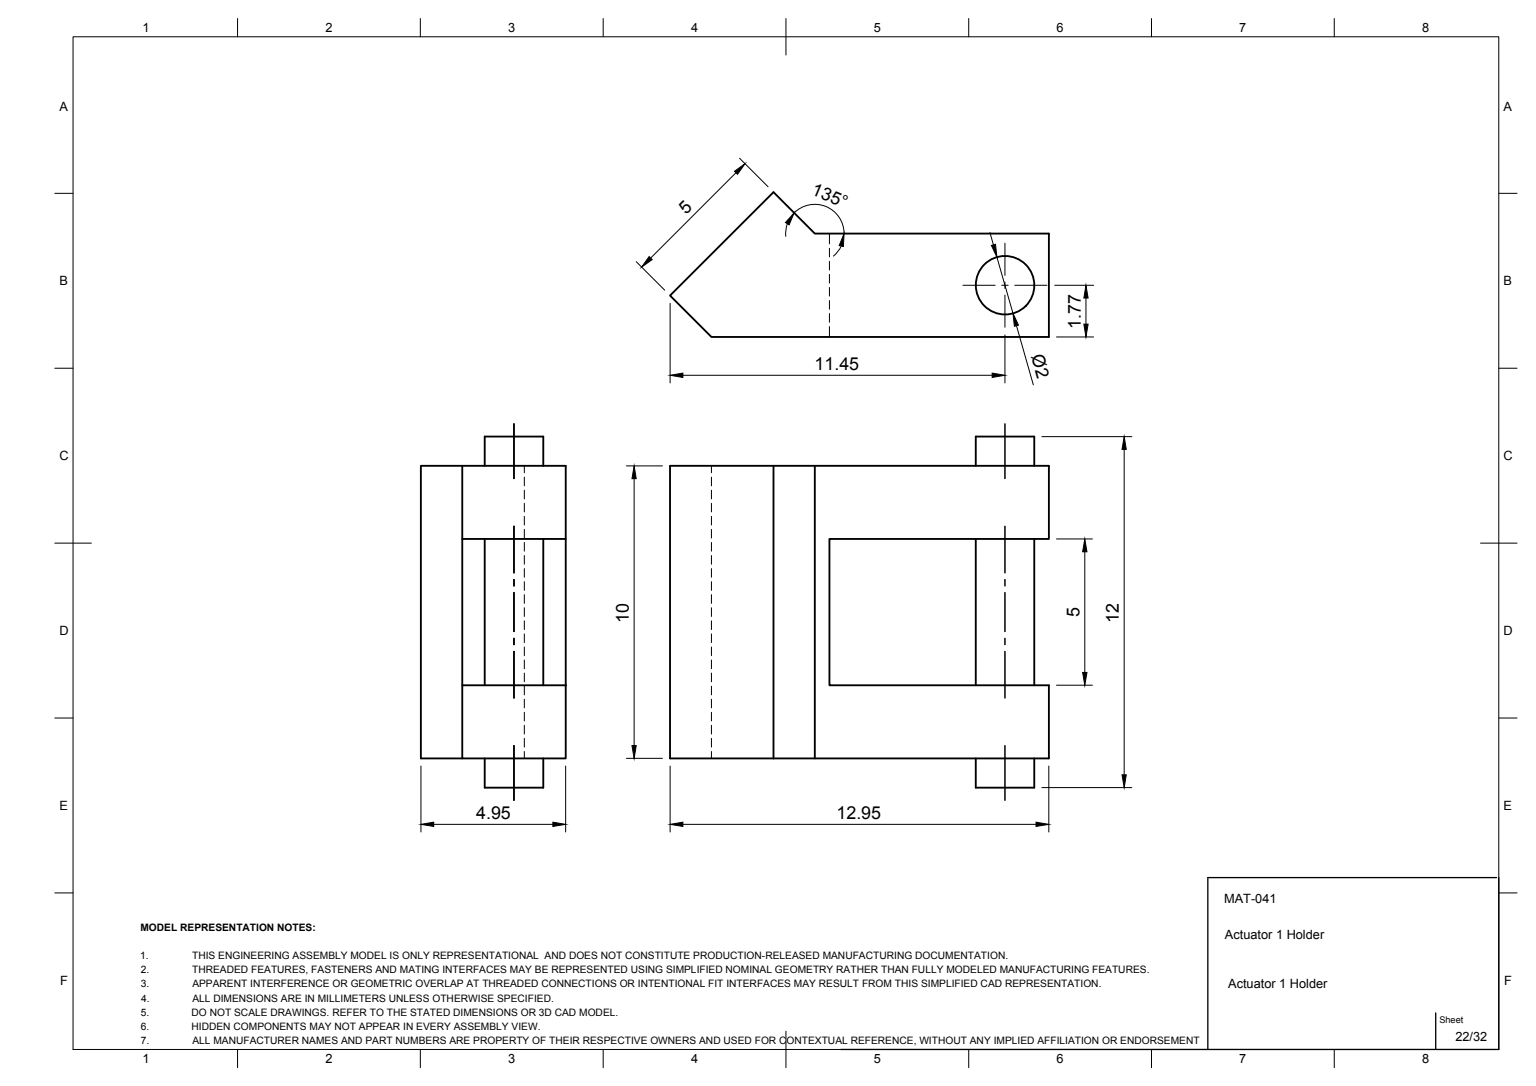
ISO-10303-21;
HEADER;
/* Generated by software containing ST-Developer
 * from STEP Tools, Inc. (www.steptools.com) 
 */

FILE_DESCRIPTION(
/* description */ ('STEP AP214'),
/* implementation_level */ '2;1');

FILE_NAME(
/* name */ 'Actuator 1 Holder.step',
/* time_stamp */ '2026-11-14T21:57:47-08:00',
/* author */ (''),
/* organization */ (''),
/* preprocessor_version */ 'ST-DEVELOPER v20.2',
/* originating_system */ 'Autodesk Translation Framework v15.17.0.0',
/* authorisation */ '');

FILE_SCHEMA (('AUTOMOTIVE_DESIGN { 1 0 10303 214 3 1 1 }'));
ENDSEC;

DATA;
#10=MECHANICAL_DESIGN_GEOMETRIC_PRESENTATION_REPRESENTATION('',(#258),#13199);
#222=SHAPE_REPRESENTATION_RELATIONSHIP('SRR','None',#13293,#240);
#240=ADVANCED_BREP_SHAPE_REPRESENTATION('',(#276),#13189);
#258=STYLED_ITEM('',(#13409),#276);
#276=MANIFOLD_SOLID_BREP('Body1',#6853);
#345=FACE_BOUND('',#2515,.T.);
#346=FACE_BOUND('',#2518,.T.);
#347=FACE_BOUND('',#2525,.T.);
#348=FACE_BOUND('',#2527,.T.);
#524=PLANE('',#7578);
#525=PLANE('',#7579);
#526=PLANE('',#7580);
#527=PLANE('',#7581);
#528=PLANE('',#7582);
#529=PLANE('',#7583);
#530=PLANE('',#7584);
#531=PLANE('',#7585);
#532=PLANE('',#7586);
#533=PLANE('',#7587);
#534=PLANE('',#7588);
#535=PLANE('',#7589);
#536=PLANE('',#7590);
#537=PLANE('',#7591);
#935=LINE('',#11859,#1453);
#936=LINE('',#11865,#1454);
#937=LINE('',#11871,#1455);
#938=LINE('',#11876,#1456);
#939=LINE('',#11878,#1457);
#940=LINE('',#11880,#1458);
#941=LINE('',#11881,#1459);
#942=LINE('',#11885,#1460);
#943=LINE('',#11887,#1461);
#944=LINE('',#11888,#1462);
#945=LINE('',#11890,#1463);
#946=LINE('',#11891,#1464);
#947=LINE('',#11894,#1465);
#948=LINE('',#11896,#1466);
#949=LINE('',#11897,#1467);
#950=LINE('',#11900,#1468);
#951=LINE('',#11902,#1469);
#952=LINE('',#11904,#1470);
#953=LINE('',#11906,#1471);
#954=LINE('',#11907,#1472);
#955=LINE('',#11909,#1473);
#956=LINE('',#11910,#1474);
#957=LINE('',#11914,#1475);
#958=LINE('',#11916,#1476);
#959=LINE('',#11918,#1477);
#960=LINE('',#11919,#1478);
#961=LINE('',#11923,#1479);
#962=LINE('',#11924,#1480);
#963=LINE('',#11926,#1481);
#964=LINE('',#11927,#1482);
#965=LINE('',#11929,#1483);
#966=LINE('',#11931,#1484);
#967=LINE('',#11933,#1485);
#1453=VECTOR('',#9176,1.);
#1454=VECTOR('',#9183,1.);
#1455=VECTOR('',#9190,1.);
#1456=VECTOR('',#9195,1000.);
#1457=VECTOR('',#9196,1000.);
#1458=VECTOR('',#9197,1000.);
#1459=VECTOR('',#9198,1000.);
#1460=VECTOR('',#9201,1000.);
#1461=VECTOR('',#9202,1000.);
#1462=VECTOR('',#9203,1000.);
#1463=VECTOR('',#9204,1000.);
#1464=VECTOR('',#9205,1000.);
#1465=VECTOR('',#9208,1000.);
#1466=VECTOR('',#9209,1000.);
#1467=VECTOR('',#9210,1000.);
#1468=VECTOR('',#9213,1000.);
#1469=VECTOR('',#9214,1000.);
#1470=VECTOR('',#9215,1000.);
#1471=VECTOR('',#9216,1000.);
#1472=VECTOR('',#9217,1000.);
#1473=VECTOR('',#9220,1000.);
#1474=VECTOR('',#9221,1000.);
#1475=VECTOR('',#9226,1000.);
#1476=VECTOR('',#9227,1000.);
#1477=VECTOR('',#9228,1000.);
#1478=VECTOR('',#9229,1000.);
#1479=VECTOR('',#9232,1000.);
#1480=VECTOR('',#9233,1000.);
#1481=VECTOR('',#9234,1000.);
#1482=VECTOR('',#9235,1000.);
#1483=VECTOR('',#9238,1000.);
#1484=VECTOR('',#9241,1000.);
#1485=VECTOR('',#9244,1000.);
#1751=CYLINDRICAL_SURFACE('',#7569,1.);
#1752=CYLINDRICAL_SURFACE('',#7572,1.);
#1753=CYLINDRICAL_SURFACE('',#7575,1.);
#2058=FACE_OUTER_BOUND('',#2510,.T.);
#2059=FACE_OUTER_BOUND('',#2511,.T.);
#2060=FACE_OUTER_BOUND('',#2512,.T.);
#2061=FACE_OUTER_BOUND('',#2513,.T.);
#2062=FACE_OUTER_BOUND('',#2514,.T.);
#2063=FACE_OUTER_BOUND('',#2516,.T.);
#2064=FACE_OUTER_BOUND('',#2517,.T.);
#2065=FACE_OUTER_BOUND('',#2519,.T.);
#2066=FACE_OUTER_BOUND('',#2520,.T.);
#2067=FACE_OUTER_BOUND('',#2521,.T.);
#2068=FACE_OUTER_BOUND('',#2522,.T.);
#2069=FACE_OUTER_BOUND('',#2523,.T.);
#2070=FACE_OUTER_BOUND('',#2524,.T.);
#2071=FACE_OUTER_BOUND('',#2526,.T.);
#2072=FACE_OUTER_BOUND('',#2528,.T.);
#2073=FACE_OUTER_BOUND('',#2529,.T.);
#2074=FACE_OUTER_BOUND('',#2530,.T.);
#2510=EDGE_LOOP('',(#5784,#5785,#5786,#5787));
#2511=EDGE_LOOP('',(#5788,#5789,#5790,#5791));
#2512=EDGE_LOOP('',(#5792,#5793,#5794,#5795));
#2513=EDGE_LOOP('',(#5796,#5797,#5798,#5799));
#2514=EDGE_LOOP('',(#5800,#5801,#5802,#5803,#5804,#5805));
#2515=EDGE_LOOP('',(#5806));
#2516=EDGE_LOOP('',(#5807,#5808,#5809,#5810));
#2517=EDGE_LOOP('',(#5811,#5812,#5813,#5814,#5815,#5816));
#2518=EDGE_LOOP('',(#5817));
#2519=EDGE_LOOP('',(#5818,#5819,#5820,#5821));
#2520=EDGE_LOOP('',(#5822,#5823,#5824,#5825));
#2521=EDGE_LOOP('',(#5826,#5827,#5828,#5829,#5830,#5831,#5832,#5833));
#2522=EDGE_LOOP('',(#5834,#5835,#5836,#5837,#5838,#5839,#5840,#5841));
#2523=EDGE_LOOP('',(#5842,#5843,#5844,#5845));
#2524=EDGE_LOOP('',(#5846,#5847,#5848,#5849));
#2525=EDGE_LOOP('',(#5850));
#2526=EDGE_LOOP('',(#5851,#5852,#5853,#5854));
#2527=EDGE_LOOP('',(#5855));
#2528=EDGE_LOOP('',(#5856,#5857,#5858,#5859));
#2529=EDGE_LOOP('',(#5860));
#2530=EDGE_LOOP('',(#5861));
#2903=CIRCLE('',#7570,1.);
#2904=CIRCLE('',#7571,1.);
#2905=CIRCLE('',#7573,1.);
#2906=CIRCLE('',#7574,1.);
#2907=CIRCLE('',#7576,1.);
#2908=CIRCLE('',#7577,1.);
#3396=VERTEX_POINT('',#11856);
#3397=VERTEX_POINT('',#11858);
#3398=VERTEX_POINT('',#11862);
#3399=VERTEX_POINT('',#11864);
#3400=VERTEX_POINT('',#11868);
#3401=VERTEX_POINT('',#11870);
#3402=VERTEX_POINT('',#11874);
#3403=VERTEX_POINT('',#11875);
#3404=VERTEX_POINT('',#11877);
#3405=VERTEX_POINT('',#11879);
#3406=VERTEX_POINT('',#11883);
#3407=VERTEX_POINT('',#11884);
#3408=VERTEX_POINT('',#11886);
#3409=VERTEX_POINT('',#11889);
#3410=VERTEX_POINT('',#11893);
#3411=VERTEX_POINT('',#11895);
#3412=VERTEX_POINT('',#11899);
#3413=VERTEX_POINT('',#11901);
#3414=VERTEX_POINT('',#11903);
#3415=VERTEX_POINT('',#11905);
#3416=VERTEX_POINT('',#11913);
#3417=VERTEX_POINT('',#11915);
#3418=VERTEX_POINT('',#11917);
#3419=VERTEX_POINT('',#11921);
#3420=VERTEX_POINT('',#11922);
#3421=VERTEX_POINT('',#11925);
#4229=EDGE_CURVE('',#3396,#3396,#2903,.T.);
#4230=EDGE_CURVE('',#3396,#3397,#935,.T.);
#4231=EDGE_CURVE('',#3397,#3397,#2904,.T.);
#4232=EDGE_CURVE('',#3398,#3398,#2905,.T.);
#4233=EDGE_CURVE('',#3398,#3399,#936,.T.);
#4234=EDGE_CURVE('',#3399,#3399,#2906,.T.);
#4235=EDGE_CURVE('',#3400,#3400,#2907,.T.);
#4236=EDGE_CURVE('',#3400,#3401,#937,.T.);
#4237=EDGE_CURVE('',#3401,#3401,#2908,.T.);
#4238=EDGE_CURVE('',#3402,#3403,#938,.T.);
#4239=EDGE_CURVE('',#3402,#3404,#939,.T.);
#4240=EDGE_CURVE('',#3404,#3405,#940,.T.);
#4241=EDGE_CURVE('',#3405,#3403,#941,.T.);
#4242=EDGE_CURVE('',#3406,#3407,#942,.T.);
#4243=EDGE_CURVE('',#3408,#3407,#943,.T.);
#4244=EDGE_CURVE('',#3405,#3408,#944,.T.);
#4245=EDGE_CURVE('',#3404,#3409,#945,.T.);
#4246=EDGE_CURVE('',#3409,#3406,#946,.T.);
#4247=EDGE_CURVE('',#3407,#3410,#947,.T.);
#4248=EDGE_CURVE('',#3411,#3410,#948,.T.);
#4249=EDGE_CURVE('',#3408,#3411,#949,.T.);
#4250=EDGE_CURVE('',#3410,#3412,#950,.T.);
#4251=EDGE_CURVE('',#3413,#3412,#951,.T.);
#4252=EDGE_CURVE('',#3414,#3413,#952,.T.);
#4253=EDGE_CURVE('',#3415,#3414,#953,.T.);
#4254=EDGE_CURVE('',#3415,#3411,#954,.T.);
#4255=EDGE_CURVE('',#3412,#3406,#955,.T.);
#4256=EDGE_CURVE('',#3413,#3409,#956,.T.);
#4257=EDGE_CURVE('',#3416,#3402,#957,.T.);
#4258=EDGE_CURVE('',#3417,#3416,#958,.T.);
#4259=EDGE_CURVE('',#3418,#3417,#959,.T.);
#4260=EDGE_CURVE('',#3414,#3418,#960,.T.);
#4261=EDGE_CURVE('',#3419,#3420,#961,.T.);
#4262=EDGE_CURVE('',#3403,#3419,#962,.T.);
#4263=EDGE_CURVE('',#3421,#3415,#963,.T.);
#4264=EDGE_CURVE('',#3420,#3421,#964,.T.);
#4265=EDGE_CURVE('',#3421,#3418,#965,.T.);
#4266=EDGE_CURVE('',#3416,#3419,#966,.T.);
#4267=EDGE_CURVE('',#3417,#3420,#967,.T.);
#5784=ORIENTED_EDGE('',*,*,#4229,.T.);
#5785=ORIENTED_EDGE('',*,*,#4230,.T.);
#5786=ORIENTED_EDGE('',*,*,#4231,.F.);
#5787=ORIENTED_EDGE('',*,*,#4230,.F.);
#5788=ORIENTED_EDGE('',*,*,#4232,.T.);
#5789=ORIENTED_EDGE('',*,*,#4233,.T.);
#5790=ORIENTED_EDGE('',*,*,#4234,.T.);
#5791=ORIENTED_EDGE('',*,*,#4233,.F.);
#5792=ORIENTED_EDGE('',*,*,#4235,.T.);
#5793=ORIENTED_EDGE('',*,*,#4236,.T.);
#5794=ORIENTED_EDGE('',*,*,#4237,.T.);
#5795=ORIENTED_EDGE('',*,*,#4236,.F.);
#5796=ORIENTED_EDGE('',*,*,#4238,.F.);
#5797=ORIENTED_EDGE('',*,*,#4239,.T.);
#5798=ORIENTED_EDGE('',*,*,#4240,.T.);
#5799=ORIENTED_EDGE('',*,*,#4241,.T.);
#5800=ORIENTED_EDGE('',*,*,#4242,.T.);
#5801=ORIENTED_EDGE('',*,*,#4243,.F.);
#5802=ORIENTED_EDGE('',*,*,#4244,.F.);
#5803=ORIENTED_EDGE('',*,*,#4240,.F.);
#5804=ORIENTED_EDGE('',*,*,#4245,.T.);
#5805=ORIENTED_EDGE('',*,*,#4246,.T.);
#5806=ORIENTED_EDGE('',*,*,#4229,.F.);
#5807=ORIENTED_EDGE('',*,*,#4247,.T.);
#5808=ORIENTED_EDGE('',*,*,#4248,.F.);
#5809=ORIENTED_EDGE('',*,*,#4249,.F.);
#5810=ORIENTED_EDGE('',*,*,#4243,.T.);
#5811=ORIENTED_EDGE('',*,*,#4250,.T.);
#5812=ORIENTED_EDGE('',*,*,#4251,.F.);
#5813=ORIENTED_EDGE('',*,*,#4252,.F.);
#5814=ORIENTED_EDGE('',*,*,#4253,.F.);
#5815=ORIENTED_EDGE('',*,*,#4254,.T.);
#5816=ORIENTED_EDGE('',*,*,#4248,.T.);
#5817=ORIENTED_EDGE('',*,*,#4234,.F.);
#5818=ORIENTED_EDGE('',*,*,#4255,.T.);
#5819=ORIENTED_EDGE('',*,*,#4246,.F.);
#5820=ORIENTED_EDGE('',*,*,#4256,.F.);
#5821=ORIENTED_EDGE('',*,*,#4251,.T.);
#5822=ORIENTED_EDGE('',*,*,#4242,.F.);
#5823=ORIENTED_EDGE('',*,*,#4255,.F.);
#5824=ORIENTED_EDGE('',*,*,#4250,.F.);
#5825=ORIENTED_EDGE('',*,*,#4247,.F.);
#5826=ORIENTED_EDGE('',*,*,#4239,.F.);
#5827=ORIENTED_EDGE('',*,*,#4257,.F.);
#5828=ORIENTED_EDGE('',*,*,#4258,.F.);
#5829=ORIENTED_EDGE('',*,*,#4259,.F.);
#5830=ORIENTED_EDGE('',*,*,#4260,.F.);
#5831=ORIENTED_EDGE('',*,*,#4252,.T.);
#5832=ORIENTED_EDGE('',*,*,#4256,.T.);
#5833=ORIENTED_EDGE('',*,*,#4245,.F.);
#5834=ORIENTED_EDGE('',*,*,#4261,.F.);
#5835=ORIENTED_EDGE('',*,*,#4262,.F.);
#5836=ORIENTED_EDGE('',*,*,#4241,.F.);
#5837=ORIENTED_EDGE('',*,*,#4244,.T.);
#5838=ORIENTED_EDGE('',*,*,#4249,.T.);
#5839=ORIENTED_EDGE('',*,*,#4254,.F.);
#5840=ORIENTED_EDGE('',*,*,#4263,.F.);
#5841=ORIENTED_EDGE('',*,*,#4264,.F.);
#5842=ORIENTED_EDGE('',*,*,#4265,.F.);
#5843=ORIENTED_EDGE('',*,*,#4263,.T.);
#5844=ORIENTED_EDGE('',*,*,#4253,.T.);
#5845=ORIENTED_EDGE('',*,*,#4260,.T.);
#5846=ORIENTED_EDGE('',*,*,#4238,.T.);
#5847=ORIENTED_EDGE('',*,*,#4262,.T.);
#5848=ORIENTED_EDGE('',*,*,#4266,.F.);
#5849=ORIENTED_EDGE('',*,*,#4257,.T.);
#5850=ORIENTED_EDGE('',*,*,#4237,.F.);
#5851=ORIENTED_EDGE('',*,*,#4265,.T.);
#5852=ORIENTED_EDGE('',*,*,#4259,.T.);
#5853=ORIENTED_EDGE('',*,*,#4267,.T.);
#5854=ORIENTED_EDGE('',*,*,#4264,.T.);
#5855=ORIENTED_EDGE('',*,*,#4235,.F.);
#5856=ORIENTED_EDGE('',*,*,#4258,.T.);
#5857=ORIENTED_EDGE('',*,*,#4266,.T.);
#5858=ORIENTED_EDGE('',*,*,#4261,.T.);
#5859=ORIENTED_EDGE('',*,*,#4267,.F.);
#5860=ORIENTED_EDGE('',*,*,#4232,.F.);
#5861=ORIENTED_EDGE('',*,*,#4231,.T.);
#6710=ADVANCED_FACE('',(#2058),#1751,.T.);
#6711=ADVANCED_FACE('',(#2059),#1752,.T.);
#6712=ADVANCED_FACE('',(#2060),#1753,.T.);
#6713=ADVANCED_FACE('',(#2061),#524,.T.);
#6714=ADVANCED_FACE('',(#2062,#345),#525,.F.);
#6715=ADVANCED_FACE('',(#2063),#526,.F.);
#6716=ADVANCED_FACE('',(#2064,#346),#527,.F.);
#6717=ADVANCED_FACE('',(#2065),#528,.F.);
#6718=ADVANCED_FACE('',(#2066),#529,.T.);
#6719=ADVANCED_FACE('',(#2067),#530,.F.);
#6720=ADVANCED_FACE('',(#2068),#531,.F.);
#6721=ADVANCED_FACE('',(#2069),#532,.T.);
#6722=ADVANCED_FACE('',(#2070,#347),#533,.F.);
#6723=ADVANCED_FACE('',(#2071,#348),#534,.F.);
#6724=ADVANCED_FACE('',(#2072),#535,.F.);
#6725=ADVANCED_FACE('',(#2073),#536,.F.);
#6726=ADVANCED_FACE('',(#2074),#537,.T.);
#6853=CLOSED_SHELL('',(#6710,#6711,#6712,#6713,#6714,#6715,#6716,#6717,
#6718,#6719,#6720,#6721,#6722,#6723,#6724,#6725,#6726));
#7568=AXIS2_PLACEMENT_3D('',#11854,#9170,#9171);
#7569=AXIS2_PLACEMENT_3D('',#11855,#9172,#9173);
#7570=AXIS2_PLACEMENT_3D('',#11857,#9174,#9175);
#7571=AXIS2_PLACEMENT_3D('',#11860,#9177,#9178);
#7572=AXIS2_PLACEMENT_3D('',#11861,#9179,#9180);
#7573=AXIS2_PLACEMENT_3D('',#11863,#9181,#9182);
#7574=AXIS2_PLACEMENT_3D('',#11866,#9184,#9185);
#7575=AXIS2_PLACEMENT_3D('',#11867,#9186,#9187);
#7576=AXIS2_PLACEMENT_3D('',#11869,#9188,#9189);
#7577=AXIS2_PLACEMENT_3D('',#11872,#9191,#9192);
#7578=AXIS2_PLACEMENT_3D('',#11873,#9193,#9194);
#7579=AXIS2_PLACEMENT_3D('',#11882,#9199,#9200);
#7580=AXIS2_PLACEMENT_3D('',#11892,#9206,#9207);
#7581=AXIS2_PLACEMENT_3D('',#11898,#9211,#9212);
#7582=AXIS2_PLACEMENT_3D('',#11908,#9218,#9219);
#7583=AXIS2_PLACEMENT_3D('',#11911,#9222,#9223);
#7584=AXIS2_PLACEMENT_3D('',#11912,#9224,#9225);
#7585=AXIS2_PLACEMENT_3D('',#11920,#9230,#9231);
#7586=AXIS2_PLACEMENT_3D('',#11928,#9236,#9237);
#7587=AXIS2_PLACEMENT_3D('',#11930,#9239,#9240);
#7588=AXIS2_PLACEMENT_3D('',#11932,#9242,#9243);
#7589=AXIS2_PLACEMENT_3D('',#11934,#9245,#9246);
#7590=AXIS2_PLACEMENT_3D('',#11935,#9247,#9248);
#7591=AXIS2_PLACEMENT_3D('',#11936,#9249,#9250);
#9170=DIRECTION('axis',(0.,0.,1.));
#9171=DIRECTION('refdir',(1.,0.,0.));
#9172=DIRECTION('center_axis',(-1.,0.,0.));
#9173=DIRECTION('ref_axis',(0.,0.,1.));
#9174=DIRECTION('center_axis',(1.,0.,0.));
#9175=DIRECTION('ref_axis',(0.,0.,1.));
#9176=DIRECTION('',(1.,0.,0.));
#9177=DIRECTION('center_axis',(1.,0.,0.));
#9178=DIRECTION('ref_axis',(0.,0.,-1.));
#9179=DIRECTION('center_axis',(-1.,0.,0.));
#9180=DIRECTION('ref_axis',(0.,0.,1.));
#9181=DIRECTION('center_axis',(1.,0.,0.));
#9182=DIRECTION('ref_axis',(0.,0.,-1.));
#9183=DIRECTION('',(1.,0.,0.));
#9184=DIRECTION('center_axis',(-1.,0.,0.));
#9185=DIRECTION('ref_axis',(0.,0.,-1.));
#9186=DIRECTION('center_axis',(-1.,0.,0.));
#9187=DIRECTION('ref_axis',(0.,0.,1.));
#9188=DIRECTION('center_axis',(1.,0.,0.));
#9189=DIRECTION('ref_axis',(0.,0.,1.));
#9190=DIRECTION('',(1.,0.,0.));
#9191=DIRECTION('center_axis',(-1.,0.,0.));
#9192=DIRECTION('ref_axis',(0.,0.,-1.));
#9193=DIRECTION('center_axis',(0.,0.707106781186547,0.707106781186548));
#9194=DIRECTION('ref_axis',(0.,-0.707106781186548,0.707106781186547));
#9195=DIRECTION('',(0.,0.707106781186548,-0.707106781186547));
#9196=DIRECTION('',(1.,0.,0.));
#9197=DIRECTION('',(0.,0.707106781186548,-0.707106781186547));
#9198=DIRECTION('',(-1.,0.,0.));
#9199=DIRECTION('center_axis',(-1.,0.,0.));
#9200=DIRECTION('ref_axis',(0.,0.,1.));
#9201=DIRECTION('',(0.,0.,-1.));
#9202=DIRECTION('',(0.,-1.,0.));
#9203=DIRECTION('',(0.,-0.707106781186547,-0.707106781186548));
#9204=DIRECTION('',(0.,-0.707106781186547,-0.707106781186548));
#9205=DIRECTION('',(0.,-1.,0.));
#9206=DIRECTION('center_axis',(0.,0.,1.));
#9207=DIRECTION('ref_axis',(1.,0.,0.));
#9208=DIRECTION('',(-1.,0.,0.));
#9209=DIRECTION('',(0.,-1.,0.));
#9210=DIRECTION('',(-1.,0.,0.));
#9211=DIRECTION('center_axis',(1.,0.,0.));
#9212=DIRECTION('ref_axis',(0.,0.,-1.));
#9213=DIRECTION('',(0.,0.,1.));
#9214=DIRECTION('',(0.,-1.,0.));
#9215=DIRECTION('',(0.,-0.707106781186547,-0.707106781186548));
#9216=DIRECTION('',(0.,-0.707106781186548,0.707106781186547));
#9217=DIRECTION('',(0.,-0.707106781186547,-0.707106781186548));
#9218=DIRECTION('center_axis',(0.,0.,-1.));
#9219=DIRECTION('ref_axis',(-1.,0.,0.));
#9220=DIRECTION('',(1.,0.,0.));
#9221=DIRECTION('',(1.,0.,0.));
#9222=DIRECTION('center_axis',(0.,-1.,0.));
#9223=DIRECTION('ref_axis',(0.,0.,-1.));
#9224=DIRECTION('center_axis',(0.,0.707106781186548,-0.707106781186547));
#9225=DIRECTION('ref_axis',(0.,0.707106781186547,0.707106781186548));
#9226=DIRECTION('',(0.,0.707106781186547,0.707106781186548));
#9227=DIRECTION('',(1.,0.,0.));
#9228=DIRECTION('',(0.,-0.707106781186547,-0.707106781186548));
#9229=DIRECTION('',(1.,0.,0.));
#9230=DIRECTION('center_axis',(0.,-0.707106781186548,0.707106781186547));
#9231=DIRECTION('ref_axis',(0.,-0.707106781186547,-0.707106781186548));
#9232=DIRECTION('',(-1.,0.,0.));
#9233=DIRECTION('',(0.,-0.707106781186547,-0.707106781186547));
#9234=DIRECTION('',(-1.,0.,0.));
#9235=DIRECTION('',(0.,0.707106781186547,0.707106781186547));
#9236=DIRECTION('center_axis',(0.,0.707106781186547,0.707106781186548));
#9237=DIRECTION('ref_axis',(0.,-0.707106781186548,0.707106781186547));
#9238=DIRECTION('',(0.,-0.707106781186548,0.707106781186547));
#9239=DIRECTION('center_axis',(1.,0.,0.));
#9240=DIRECTION('ref_axis',(0.,0.,-1.));
#9241=DIRECTION('',(0.,0.707106781186548,-0.707106781186548));
#9242=DIRECTION('center_axis',(-1.,0.,0.));
#9243=DIRECTION('ref_axis',(0.,0.,1.));
#9244=DIRECTION('',(0.,0.707106781186548,-0.707106781186548));
#9245=DIRECTION('center_axis',(0.,-0.707106781186548,-0.707106781186548));
#9246=DIRECTION('ref_axis',(0.,0.707106781186548,-0.707106781186548));
#9247=DIRECTION('center_axis',(1.,0.,0.));
#9248=DIRECTION('ref_axis',(0.,0.,-1.));
#9249=DIRECTION('center_axis',(1.,0.,0.));
#9250=DIRECTION('ref_axis',(0.,0.,-1.));
#11854=CARTESIAN_POINT('',(0.,0.,0.));
#11855=CARTESIAN_POINT('Origin',(6.,7.84619407771256,5.84619407771256));
#11856=CARTESIAN_POINT('',(5.,7.84619407771256,4.84619407771256));
#11857=CARTESIAN_POINT('Origin',(5.,7.84619407771256,5.84619407771256));
#11858=CARTESIAN_POINT('',(6.,7.84619407771256,4.84619407771256));
#11859=CARTESIAN_POINT('',(6.,7.84619407771256,4.84619407771256));
#11860=CARTESIAN_POINT('Origin',(6.,7.84619407771256,5.84619407771256));
#11861=CARTESIAN_POINT('Origin',(6.,7.84619407771256,5.84619407771256));
#11862=CARTESIAN_POINT('',(-6.,7.84619407771256,4.84619407771256));
#11863=CARTESIAN_POINT('Origin',(-6.,7.84619407771256,5.84619407771256));
#11864=CARTESIAN_POINT('',(-5.,7.84619407771256,4.84619407771256));
#11865=CARTESIAN_POINT('',(6.,7.84619407771256,4.84619407771256));
#11866=CARTESIAN_POINT('Origin',(-5.,7.84619407771256,5.84619407771256));
#11867=CARTESIAN_POINT('Origin',(6.,7.84619407771256,5.84619407771256));
#11868=CARTESIAN_POINT('',(-2.5,7.84619407771256,4.84619407771256));
#11869=CARTESIAN_POINT('Origin',(-2.5,7.84619407771256,5.84619407771256));
#11870=CARTESIAN_POINT('',(2.5,7.84619407771256,4.84619407771256));
#11871=CARTESIAN_POINT('',(6.,7.84619407771256,4.84619407771256));
#11872=CARTESIAN_POINT('Origin',(2.5,7.84619407771256,5.84619407771256));
#11873=CARTESIAN_POINT('Origin',(0.,7.90685424949238,7.90685424949238));
#11874=CARTESIAN_POINT('',(2.5,7.65685424949238,8.15685424949238));
#11875=CARTESIAN_POINT('',(2.5,10.1568542494924,5.65685424949238));
#11876=CARTESIAN_POINT('',(2.5,7.90685424949238,7.90685424949238));
#11877=CARTESIAN_POINT('',(5.,7.65685424949238,8.15685424949238));
#11878=CARTESIAN_POINT('',(-5.,7.65685424949238,8.15685424949238));
#11879=CARTESIAN_POINT('',(5.,10.1568542494924,5.65685424949238));
#11880=CARTESIAN_POINT('',(5.,7.65685424949238,8.15685424949238));
#11881=CARTESIAN_POINT('',(5.,10.1568542494924,5.65685424949238));
#11882=CARTESIAN_POINT('Origin',(5.,2.,2.5));
#11883=CARTESIAN_POINT('',(5.,0.,2.5));
#11884=CARTESIAN_POINT('',(5.,0.,-2.5));
#11885=CARTESIAN_POINT('',(5.,0.,2.5));
#11886=CARTESIAN_POINT('',(5.,2.,-2.5));
#11887=CARTESIAN_POINT('',(5.,2.,-2.5));
#11888=CARTESIAN_POINT('',(5.,10.1568542494924,5.65685424949238));
#11889=CARTESIAN_POINT('',(5.,2.,2.5));
#11890=CARTESIAN_POINT('',(5.,7.65685424949238,8.15685424949238));
#11891=CARTESIAN_POINT('',(5.,2.,2.5));
#11892=CARTESIAN_POINT('Origin',(-5.,2.,-2.5));
#11893=CARTESIAN_POINT('',(-5.,0.,-2.5));
#11894=CARTESIAN_POINT('',(-5.,0.,-2.5));
#11895=CARTESIAN_POINT('',(-5.,2.,-2.5));
#11896=CARTESIAN_POINT('',(-5.,2.,-2.5));
#11897=CARTESIAN_POINT('',(-5.,2.,-2.5));
#11898=CARTESIAN_POINT('Origin',(-5.,2.,2.5));
#11899=CARTESIAN_POINT('',(-5.,0.,2.5));
#11900=CARTESIAN_POINT('',(-5.,0.,2.5));
#11901=CARTESIAN_POINT('',(-5.,2.,2.5));
#11902=CARTESIAN_POINT('',(-5.,2.,2.5));
#11903=CARTESIAN_POINT('',(-5.,7.65685424949238,8.15685424949238));
#11904=CARTESIAN_POINT('',(-5.,7.65685424949238,8.15685424949238));
#11905=CARTESIAN_POINT('',(-5.,10.1568542494924,5.65685424949238));
#11906=CARTESIAN_POINT('',(-5.,10.1568542494924,5.65685424949238));
#11907=CARTESIAN_POINT('',(-5.,10.1568542494924,5.65685424949238));
#11908=CARTESIAN_POINT('Origin',(-5.,2.,2.5));
#11909=CARTESIAN_POINT('',(-5.,0.,2.5));
#11910=CARTESIAN_POINT('',(-5.,2.,2.5));
#11911=CARTESIAN_POINT('Origin',(0.,0.,0.));
#11912=CARTESIAN_POINT('Origin',(-5.,7.65685424949238,8.15685424949238));
#11913=CARTESIAN_POINT('',(2.5,2.35355339059327,2.85355339059327));
#11914=CARTESIAN_POINT('',(2.5,12.9601551083915,13.4601551083915));
#11915=CARTESIAN_POINT('',(-2.5,2.35355339059327,2.85355339059327));
#11916=CARTESIAN_POINT('',(-2.5,2.35355339059327,2.85355339059327));
#11917=CARTESIAN_POINT('',(-2.5,7.65685424949238,8.15685424949238));
#11918=CARTESIAN_POINT('',(-2.5,12.9601551083915,13.4601551083915));
#11919=CARTESIAN_POINT('',(-5.,7.65685424949238,8.15685424949238));
#11920=CARTESIAN_POINT('Origin',(5.,10.1568542494924,5.65685424949238));
#11921=CARTESIAN_POINT('',(2.5,4.85355339059327,0.353553390593271));
#11922=CARTESIAN_POINT('',(-2.5,4.85355339059327,0.353553390593271));
#11923=CARTESIAN_POINT('',(-2.5,4.85355339059327,0.353553390593271));
#11924=CARTESIAN_POINT('',(2.5,15.4601551083915,10.9601551083915));
#11925=CARTESIAN_POINT('',(-2.5,10.1568542494924,5.65685424949238));
#11926=CARTESIAN_POINT('',(5.,10.1568542494924,5.65685424949238));
#11927=CARTESIAN_POINT('',(-2.5,15.4601551083915,10.9601551083915));
#11928=CARTESIAN_POINT('Origin',(0.,7.90685424949238,7.90685424949238));
#11929=CARTESIAN_POINT('',(-2.5,7.90685424949238,7.90685424949238));
#11930=CARTESIAN_POINT('Origin',(2.5,1.77981522089254,24.6404949958904));
#11931=CARTESIAN_POINT('',(2.5,-8.82678649690568,14.0338932780922));
#11932=CARTESIAN_POINT('Origin',(-2.5,1.77981522089254,24.6404949958904));
#11933=CARTESIAN_POINT('',(-2.5,-8.82678649690568,14.0338932780922));
#11934=CARTESIAN_POINT('Origin',(-2.5,-8.82678649690568,14.0338932780922));
#11935=CARTESIAN_POINT('Origin',(-6.,7.84619407771256,5.84619407771256));
#11936=CARTESIAN_POINT('Origin',(6.,7.84619407771256,5.84619407771256));
#13163=UNCERTAINTY_MEASURE_WITH_UNIT(LENGTH_MEASURE(0.01),#13200,
'DISTANCE_ACCURACY_VALUE',
'Maximum model space distance between geometric entities at asserted c
onnectivities');
#13173=UNCERTAINTY_MEASURE_WITH_UNIT(LENGTH_MEASURE(0.01),#13200,
'DISTANCE_ACCURACY_VALUE',
'Maximum model space distance between geometric entities at asserted c
onnectivities');
#13189=(
GEOMETRIC_REPRESENTATION_CONTEXT(3)
GLOBAL_UNCERTAINTY_ASSIGNED_CONTEXT((#13163))
GLOBAL_UNIT_ASSIGNED_CONTEXT((#13200,#13202,#13203))
REPRESENTATION_CONTEXT('','3D')
);
#13199=(
GEOMETRIC_REPRESENTATION_CONTEXT(3)
GLOBAL_UNCERTAINTY_ASSIGNED_CONTEXT((#13173))
GLOBAL_UNIT_ASSIGNED_CONTEXT((#13200,#13202,#13203))
REPRESENTATION_CONTEXT('','3D')
);
#13200=(
LENGTH_UNIT()
NAMED_UNIT(*)
SI_UNIT(.MILLI.,.METRE.)
);
#13202=(
NAMED_UNIT(*)
PLANE_ANGLE_UNIT()
SI_UNIT($,.RADIAN.)
);
#13203=(
NAMED_UNIT(*)
SI_UNIT($,.STERADIAN.)
SOLID_ANGLE_UNIT()
);
#13219=SHAPE_DEFINITION_REPRESENTATION(#13248,#13293);
#13248=PRODUCT_DEFINITION_SHAPE('',$,#13319);
#13293=SHAPE_REPRESENTATION('',(#7568),#13189);
#13303=PRODUCT_DEFINITION_CONTEXT('part definition',#13380,'design');
#13319=PRODUCT_DEFINITION('Actuator 1 Holder','Actuator 1 Holder',#13344,
#13303);
#13344=PRODUCT_DEFINITION_FORMATION('',$,#13397);
#13380=APPLICATION_CONTEXT(
'Core Data for Automotive Mechanical Design Process');
#13381=PRODUCT_CONTEXT('part definition',#13380,'mechanical');
#13397=PRODUCT('Actuator 1 Holder','Actuator 1 Holder',$,(#13381));
#13409=PRESENTATION_STYLE_ASSIGNMENT((#13414));
#13414=SURFACE_STYLE_USAGE(.BOTH.,#13419);
#13419=SURFACE_SIDE_STYLE('',(#13424));
#13424=SURFACE_STYLE_FILL_AREA(#13429);
#13429=FILL_AREA_STYLE('Opaque(61,176,222)',(#13434));
#13434=FILL_AREA_STYLE_COLOUR('Opaque(61,176,222)',#13439);
#13439=COLOUR_RGB('Opaque(61,176,222)',0.23921568627451,0.690196078431373,
0.870588235294118);
ENDSEC;
END-ISO-10303-21;
